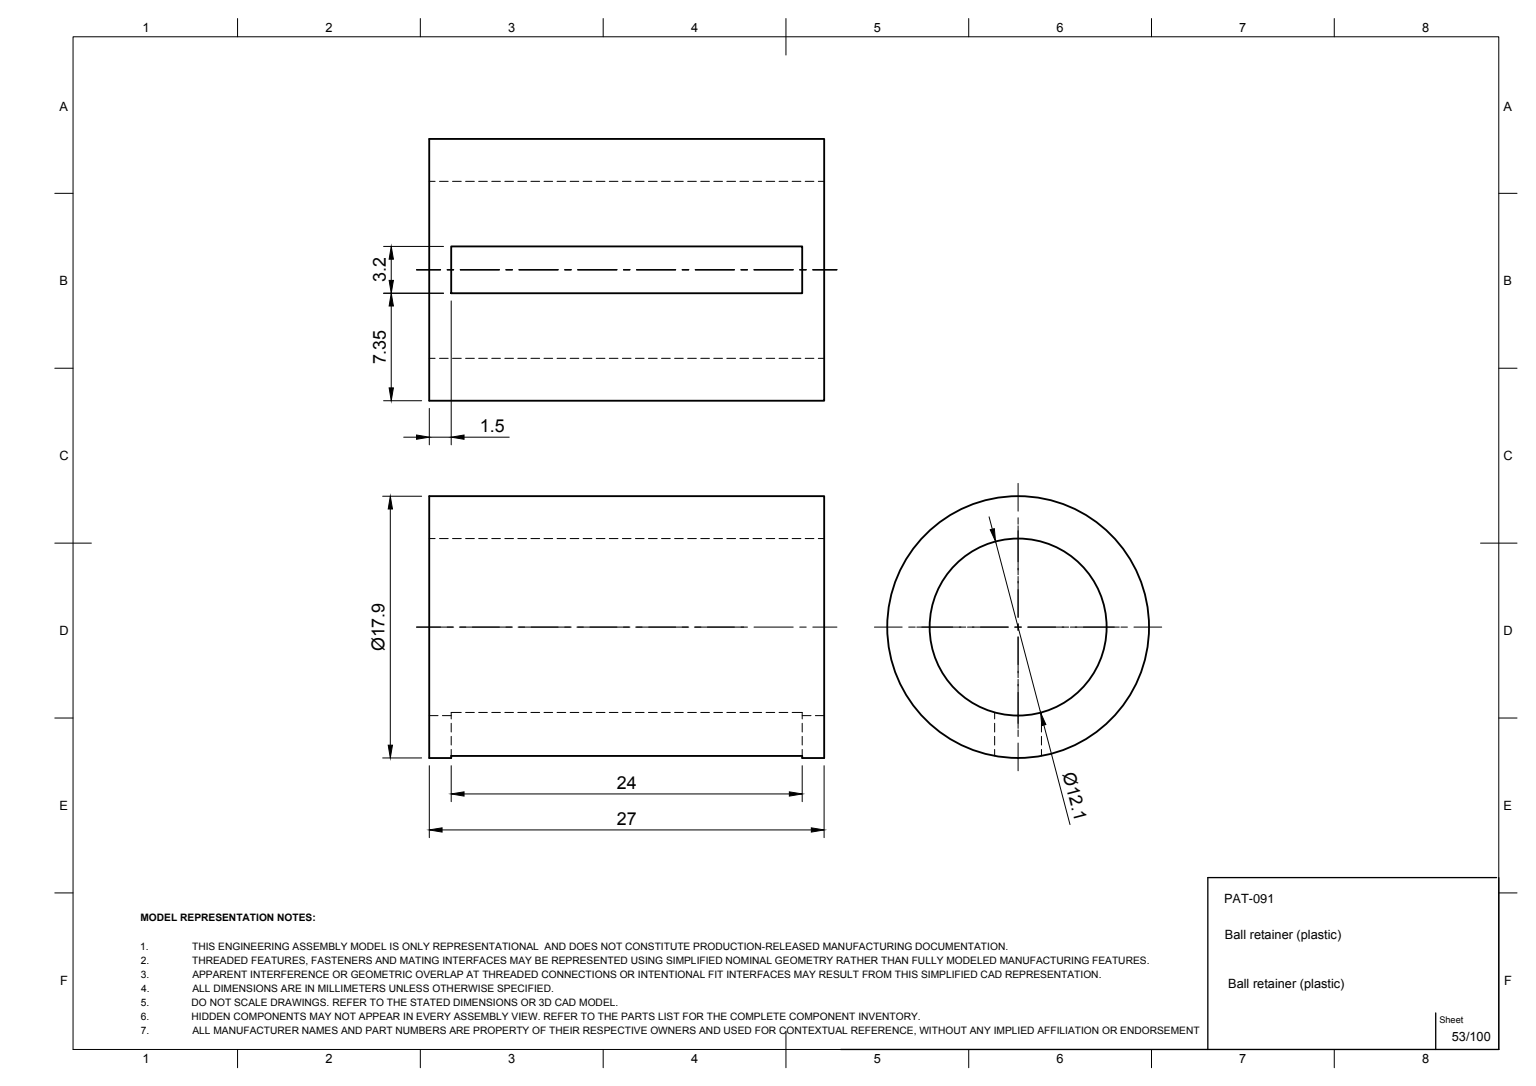
ISO-10303-21;
HEADER;
/* Generated by software containing ST-Developer
 * from STEP Tools, Inc. (www.steptools.com) 
 */

FILE_DESCRIPTION(
/* description */ ('PAT-091'),
/* implementation_level */ '2;1');

FILE_NAME(
/* name */ 'Ball retainer (plastic).step',
/* time_stamp */ '2026-10-27T15:34:44-07:00',
/* author */ (''),
/* organization */ (''),
/* preprocessor_version */ 'ST-DEVELOPER v20.2',
/* originating_system */ 'Autodesk Translation Framework v15.17.0.0',
/* authorisation */ '');

FILE_SCHEMA (('AUTOMOTIVE_DESIGN { 1 0 10303 214 3 1 1 }'));
ENDSEC;

DATA;
#10=MECHANICAL_DESIGN_GEOMETRIC_PRESENTATION_REPRESENTATION('',(#1025),#25100);
#805=SHAPE_REPRESENTATION_RELATIONSHIP('SRR','None',#25570,#915);
#915=ADVANCED_BREP_SHAPE_REPRESENTATION('',(#1147),#25040);
#1025=STYLED_ITEM('',(#26184),#1147);
#1147=MANIFOLD_SOLID_BREP('Body1',#13304);
#1479=FACE_BOUND('',#3579,.T.);
#1480=FACE_BOUND('',#3581,.T.);
#1481=FACE_BOUND('',#3583,.T.);
#1482=FACE_BOUND('',#3585,.T.);
#1880=PLANE('',#15452);
#1881=PLANE('',#15455);
#1882=PLANE('',#15456);
#1883=PLANE('',#15459);
#1884=PLANE('',#15460);
#1885=PLANE('',#15465);
#2492=FACE_OUTER_BOUND('',#3574,.T.);
#2493=FACE_OUTER_BOUND('',#3575,.T.);
#2494=FACE_OUTER_BOUND('',#3576,.T.);
#2495=FACE_OUTER_BOUND('',#3577,.T.);
#2496=FACE_OUTER_BOUND('',#3578,.T.);
#2497=FACE_OUTER_BOUND('',#3580,.T.);
#2498=FACE_OUTER_BOUND('',#3582,.T.);
#2499=FACE_OUTER_BOUND('',#3584,.T.);
#3574=EDGE_LOOP('',(#10692,#10693,#10694,#10695));
#3575=EDGE_LOOP('',(#10696,#10697,#10698,#10699));
#3576=EDGE_LOOP('',(#10700,#10701,#10702,#10703));
#3577=EDGE_LOOP('',(#10704,#10705,#10706,#10707));
#3578=EDGE_LOOP('',(#10708));
#3579=EDGE_LOOP('',(#10709));
#3580=EDGE_LOOP('',(#10710,#10711,#10712,#10713));
#3581=EDGE_LOOP('',(#10714,#10715,#10716,#10717));
#3582=EDGE_LOOP('',(#10718));
#3583=EDGE_LOOP('',(#10719));
#3584=EDGE_LOOP('',(#10720,#10721,#10722,#10723));
#3585=EDGE_LOOP('',(#10724,#10725,#10726,#10727));
#4603=LINE('',#22952,#5343);
#4604=LINE('',#22955,#5344);
#4605=LINE('',#22958,#5345);
#4606=LINE('',#22960,#5346);
#4607=LINE('',#22961,#5347);
#4608=LINE('',#22967,#5348);
#4609=LINE('',#22969,#5349);
#4610=LINE('',#22970,#5350);
#4611=LINE('',#22979,#5351);
#4612=LINE('',#22984,#5352);
#5343=VECTOR('',#18685,1.);
#5344=VECTOR('',#18688,1.);
#5345=VECTOR('',#18691,1.);
#5346=VECTOR('',#18692,1.);
#5347=VECTOR('',#18693,1.);
#5348=VECTOR('',#18700,1.);
#5349=VECTOR('',#18703,1.);
#5350=VECTOR('',#18704,1.);
#5351=VECTOR('',#18715,0.895);
#5352=VECTOR('',#18722,0.605);
#5981=CIRCLE('',#15453,0.895);
#5982=CIRCLE('',#15454,0.605);
#5983=CIRCLE('',#15457,0.895);
#5984=CIRCLE('',#15458,0.605);
#5985=CIRCLE('',#15461,0.895);
#5986=CIRCLE('',#15462,0.605);
#5987=CIRCLE('',#15464,0.895);
#5988=CIRCLE('',#15466,0.605);
#6954=VERTEX_POINT('',#22948);
#6955=VERTEX_POINT('',#22949);
#6956=VERTEX_POINT('',#22951);
#6957=VERTEX_POINT('',#22953);
#6958=VERTEX_POINT('',#22957);
#6959=VERTEX_POINT('',#22959);
#6960=VERTEX_POINT('',#22963);
#6961=VERTEX_POINT('',#22965);
#6962=VERTEX_POINT('',#22972);
#6963=VERTEX_POINT('',#22974);
#6964=VERTEX_POINT('',#22977);
#6965=VERTEX_POINT('',#22981);
#8281=EDGE_CURVE('',#6954,#6955,#5981,.T.);
#8282=EDGE_CURVE('',#6956,#6954,#4603,.T.);
#8283=EDGE_CURVE('',#6957,#6956,#5982,.T.);
#8284=EDGE_CURVE('',#6955,#6957,#4604,.T.);
#8285=EDGE_CURVE('',#6955,#6958,#4605,.T.);
#8286=EDGE_CURVE('',#6959,#6957,#4606,.T.);
#8287=EDGE_CURVE('',#6959,#6958,#4607,.T.);
#8288=EDGE_CURVE('',#6958,#6960,#5983,.T.);
#8289=EDGE_CURVE('',#6961,#6959,#5984,.T.);
#8290=EDGE_CURVE('',#6960,#6961,#4608,.T.);
#8291=EDGE_CURVE('',#6960,#6954,#4609,.T.);
#8292=EDGE_CURVE('',#6956,#6961,#4610,.T.);
#8293=EDGE_CURVE('',#6962,#6962,#5985,.T.);
#8294=EDGE_CURVE('',#6963,#6963,#5986,.T.);
#8295=EDGE_CURVE('',#6964,#6964,#5987,.T.);
#8296=EDGE_CURVE('',#6964,#6962,#4611,.T.);
#8297=EDGE_CURVE('',#6965,#6965,#5988,.T.);
#8298=EDGE_CURVE('',#6965,#6963,#4612,.T.);
#10692=ORIENTED_EDGE('',*,*,#8281,.F.);
#10693=ORIENTED_EDGE('',*,*,#8282,.F.);
#10694=ORIENTED_EDGE('',*,*,#8283,.F.);
#10695=ORIENTED_EDGE('',*,*,#8284,.F.);
#10696=ORIENTED_EDGE('',*,*,#8285,.F.);
#10697=ORIENTED_EDGE('',*,*,#8284,.T.);
#10698=ORIENTED_EDGE('',*,*,#8286,.F.);
#10699=ORIENTED_EDGE('',*,*,#8287,.T.);
#10700=ORIENTED_EDGE('',*,*,#8288,.F.);
#10701=ORIENTED_EDGE('',*,*,#8287,.F.);
#10702=ORIENTED_EDGE('',*,*,#8289,.F.);
#10703=ORIENTED_EDGE('',*,*,#8290,.F.);
#10704=ORIENTED_EDGE('',*,*,#8291,.F.);
#10705=ORIENTED_EDGE('',*,*,#8290,.T.);
#10706=ORIENTED_EDGE('',*,*,#8292,.F.);
#10707=ORIENTED_EDGE('',*,*,#8282,.T.);
#10708=ORIENTED_EDGE('',*,*,#8293,.F.);
#10709=ORIENTED_EDGE('',*,*,#8294,.T.);
#10710=ORIENTED_EDGE('',*,*,#8295,.F.);
#10711=ORIENTED_EDGE('',*,*,#8296,.T.);
#10712=ORIENTED_EDGE('',*,*,#8293,.T.);
#10713=ORIENTED_EDGE('',*,*,#8296,.F.);
#10714=ORIENTED_EDGE('',*,*,#8288,.T.);
#10715=ORIENTED_EDGE('',*,*,#8291,.T.);
#10716=ORIENTED_EDGE('',*,*,#8281,.T.);
#10717=ORIENTED_EDGE('',*,*,#8285,.T.);
#10718=ORIENTED_EDGE('',*,*,#8295,.T.);
#10719=ORIENTED_EDGE('',*,*,#8297,.F.);
#10720=ORIENTED_EDGE('',*,*,#8297,.T.);
#10721=ORIENTED_EDGE('',*,*,#8298,.T.);
#10722=ORIENTED_EDGE('',*,*,#8294,.F.);
#10723=ORIENTED_EDGE('',*,*,#8298,.F.);
#10724=ORIENTED_EDGE('',*,*,#8289,.T.);
#10725=ORIENTED_EDGE('',*,*,#8286,.T.);
#10726=ORIENTED_EDGE('',*,*,#8283,.T.);
#10727=ORIENTED_EDGE('',*,*,#8292,.T.);
#12256=CYLINDRICAL_SURFACE('',#15463,0.895);
#12257=CYLINDRICAL_SURFACE('',#15467,0.605);
#12859=ADVANCED_FACE('',(#2492),#1880,.F.);
#12860=ADVANCED_FACE('',(#2493),#1881,.F.);
#12861=ADVANCED_FACE('',(#2494),#1882,.F.);
#12862=ADVANCED_FACE('',(#2495),#1883,.F.);
#12863=ADVANCED_FACE('',(#2496,#1479),#1884,.T.);
#12864=ADVANCED_FACE('',(#2497,#1480),#12256,.T.);
#12865=ADVANCED_FACE('',(#2498,#1481),#1885,.T.);
#12866=ADVANCED_FACE('',(#2499,#1482),#12257,.F.);
#13304=CLOSED_SHELL('',(#12859,#12860,#12861,#12862,#12863,#12864,#12865,
#12866));
#15451=AXIS2_PLACEMENT_3D('',#22946,#18679,#18680);
#15452=AXIS2_PLACEMENT_3D('',#22947,#18681,#18682);
#15453=AXIS2_PLACEMENT_3D('',#22950,#18683,#18684);
#15454=AXIS2_PLACEMENT_3D('',#22954,#18686,#18687);
#15455=AXIS2_PLACEMENT_3D('',#22956,#18689,#18690);
#15456=AXIS2_PLACEMENT_3D('',#22962,#18694,#18695);
#15457=AXIS2_PLACEMENT_3D('',#22964,#18696,#18697);
#15458=AXIS2_PLACEMENT_3D('',#22966,#18698,#18699);
#15459=AXIS2_PLACEMENT_3D('',#22968,#18701,#18702);
#15460=AXIS2_PLACEMENT_3D('',#22971,#18705,#18706);
#15461=AXIS2_PLACEMENT_3D('',#22973,#18707,#18708);
#15462=AXIS2_PLACEMENT_3D('',#22975,#18709,#18710);
#15463=AXIS2_PLACEMENT_3D('',#22976,#18711,#18712);
#15464=AXIS2_PLACEMENT_3D('',#22978,#18713,#18714);
#15465=AXIS2_PLACEMENT_3D('',#22980,#18716,#18717);
#15466=AXIS2_PLACEMENT_3D('',#22982,#18718,#18719);
#15467=AXIS2_PLACEMENT_3D('',#22983,#18720,#18721);
#18679=DIRECTION('axis',(0.,0.,1.));
#18680=DIRECTION('refdir',(1.,0.,0.));
#18681=DIRECTION('center_axis',(0.,1.,0.));
#18682=DIRECTION('ref_axis',(0.,0.,1.));
#18683=DIRECTION('center_axis',(0.,1.,0.));
#18684=DIRECTION('ref_axis',(1.,0.,0.));
#18685=DIRECTION('',(1.,0.,0.));
#18686=DIRECTION('center_axis',(0.,-1.,0.));
#18687=DIRECTION('ref_axis',(1.,0.,0.));
#18688=DIRECTION('',(-1.,0.,0.));
#18689=DIRECTION('center_axis',(0.,0.,-1.));
#18690=DIRECTION('ref_axis',(-1.,0.,0.));
#18691=DIRECTION('',(0.,-1.,0.));
#18692=DIRECTION('',(0.,1.,0.));
#18693=DIRECTION('',(1.,0.,0.));
#18694=DIRECTION('center_axis',(0.,-1.,0.));
#18695=DIRECTION('ref_axis',(0.,0.,-1.));
#18696=DIRECTION('center_axis',(0.,-1.,0.));
#18697=DIRECTION('ref_axis',(1.,0.,0.));
#18698=DIRECTION('center_axis',(0.,1.,0.));
#18699=DIRECTION('ref_axis',(1.,0.,0.));
#18700=DIRECTION('',(-1.,0.,0.));
#18701=DIRECTION('center_axis',(0.,0.,1.));
#18702=DIRECTION('ref_axis',(1.,0.,0.));
#18703=DIRECTION('',(0.,1.,0.));
#18704=DIRECTION('',(0.,-1.,0.));
#18705=DIRECTION('center_axis',(0.,1.,0.));
#18706=DIRECTION('ref_axis',(0.,0.,1.));
#18707=DIRECTION('center_axis',(0.,-1.,0.));
#18708=DIRECTION('ref_axis',(1.,0.,0.));
#18709=DIRECTION('center_axis',(0.,-1.,0.));
#18710=DIRECTION('ref_axis',(1.,0.,0.));
#18711=DIRECTION('center_axis',(0.,-1.,0.));
#18712=DIRECTION('ref_axis',(1.,0.,0.));
#18713=DIRECTION('center_axis',(0.,-1.,0.));
#18714=DIRECTION('ref_axis',(1.,0.,0.));
#18715=DIRECTION('',(0.,1.,0.));
#18716=DIRECTION('center_axis',(0.,-1.,0.));
#18717=DIRECTION('ref_axis',(0.,0.,-1.));
#18718=DIRECTION('center_axis',(0.,-1.,0.));
#18719=DIRECTION('ref_axis',(1.,0.,0.));
#18720=DIRECTION('center_axis',(0.,-1.,0.));
#18721=DIRECTION('ref_axis',(1.,0.,0.));
#18722=DIRECTION('',(0.,1.,0.));
#22946=CARTESIAN_POINT('',(0.,0.,0.));
#22947=CARTESIAN_POINT('Origin',(0.75,1.2,0.));
#22948=CARTESIAN_POINT('',(0.880582193778639,1.2,0.16));
#22949=CARTESIAN_POINT('',(0.880582193778639,1.2,-0.16));
#22950=CARTESIAN_POINT('Origin',(0.,1.2,0.));
#22951=CARTESIAN_POINT('',(0.583459510163302,1.2,0.16));
#22952=CARTESIAN_POINT('',(0.57,1.2,0.16));
#22953=CARTESIAN_POINT('',(0.583459510163302,1.2,-0.16));
#22954=CARTESIAN_POINT('Origin',(0.,1.2,0.));
#22955=CARTESIAN_POINT('',(0.93,1.2,-0.16));
#22956=CARTESIAN_POINT('Origin',(0.93,0.,-0.16));
#22957=CARTESIAN_POINT('',(0.880582193778639,-1.2,-0.16));
#22958=CARTESIAN_POINT('',(0.880582193778639,0.,-0.16));
#22959=CARTESIAN_POINT('',(0.583459510163302,-1.2,-0.16));
#22960=CARTESIAN_POINT('',(0.583459510163302,0.,-0.16));
#22961=CARTESIAN_POINT('',(0.93,-1.2,-0.16));
#22962=CARTESIAN_POINT('Origin',(0.75,-1.2,0.));
#22963=CARTESIAN_POINT('',(0.880582193778639,-1.2,0.16));
#22964=CARTESIAN_POINT('Origin',(0.,-1.2,0.));
#22965=CARTESIAN_POINT('',(0.583459510163302,-1.2,0.16));
#22966=CARTESIAN_POINT('Origin',(0.,-1.2,0.));
#22967=CARTESIAN_POINT('',(0.57,-1.2,0.16));
#22968=CARTESIAN_POINT('Origin',(0.57,0.,0.16));
#22969=CARTESIAN_POINT('',(0.880582193778639,0.,0.16));
#22970=CARTESIAN_POINT('',(0.583459510163302,0.,0.16));
#22971=CARTESIAN_POINT('Origin',(0.895,1.35,0.));
#22972=CARTESIAN_POINT('',(-0.895,1.35,-1.09605888523688E-16));
#22973=CARTESIAN_POINT('Origin',(0.,1.35,0.));
#22974=CARTESIAN_POINT('',(-0.605,1.35,-7.40911313484149E-17));
#22975=CARTESIAN_POINT('Origin',(0.,1.35,0.));
#22976=CARTESIAN_POINT('Origin',(0.,0.,0.));
#22977=CARTESIAN_POINT('',(-0.895,-1.35,-1.09605888523688E-16));
#22978=CARTESIAN_POINT('Origin',(0.,-1.35,0.));
#22979=CARTESIAN_POINT('',(-0.895,0.,-1.09605888523688E-16));
#22980=CARTESIAN_POINT('Origin',(0.605,-1.35,0.));
#22981=CARTESIAN_POINT('',(-0.605,-1.35,-7.40911313484149E-17));
#22982=CARTESIAN_POINT('Origin',(0.,-1.35,0.));
#22983=CARTESIAN_POINT('Origin',(0.,0.,0.));
#22984=CARTESIAN_POINT('',(-0.605,0.,-7.40911313484149E-17));
#24919=UNCERTAINTY_MEASURE_WITH_UNIT(LENGTH_MEASURE(0.001),#25101,
'DISTANCE_ACCURACY_VALUE',
'Maximum model space distance between geometric entities at asserted c
onnectivities');
#24979=UNCERTAINTY_MEASURE_WITH_UNIT(LENGTH_MEASURE(0.001),#25101,
'DISTANCE_ACCURACY_VALUE',
'Maximum model space distance between geometric entities at asserted c
onnectivities');
#25040=(
GEOMETRIC_REPRESENTATION_CONTEXT(3)
GLOBAL_UNCERTAINTY_ASSIGNED_CONTEXT((#24919))
GLOBAL_UNIT_ASSIGNED_CONTEXT((#25101,#25103,#25104))
REPRESENTATION_CONTEXT('','3D')
);
#25100=(
GEOMETRIC_REPRESENTATION_CONTEXT(3)
GLOBAL_UNCERTAINTY_ASSIGNED_CONTEXT((#24979))
GLOBAL_UNIT_ASSIGNED_CONTEXT((#25101,#25103,#25104))
REPRESENTATION_CONTEXT('','3D')
);
#25101=(
LENGTH_UNIT()
NAMED_UNIT(*)
SI_UNIT(.CENTI.,.METRE.)
);
#25103=(
NAMED_UNIT(*)
PLANE_ANGLE_UNIT()
SI_UNIT($,.RADIAN.)
);
#25104=(
NAMED_UNIT(*)
SI_UNIT($,.STERADIAN.)
SOLID_ANGLE_UNIT()
);
#25165=SHAPE_DEFINITION_REPRESENTATION(#25285,#25570);
#25285=PRODUCT_DEFINITION_SHAPE('',$,#25691);
#25570=SHAPE_REPRESENTATION('',(#15451),#25040);
#25630=PRODUCT_DEFINITION_CONTEXT('part definition',#25992,'design');
#25691=PRODUCT_DEFINITION('Ball retainer (plastic)',
'Ball retainer (plastic)',#25811,#25630);
#25811=PRODUCT_DEFINITION_FORMATION('',$,#26054);
#25992=APPLICATION_CONTEXT(
'Core Data for Automotive Mechanical Design Process');
#25993=PRODUCT_CONTEXT('part definition',#25992,'mechanical');
#26054=PRODUCT('Ball retainer (plastic)','Ball retainer (plastic)',
'Ball retainer (plastic)',(#25993));
#26178=COLOUR_RGB('Sky Blue',0.24,0.69,0.87);
#26179=FILL_AREA_STYLE_COLOUR('',#26178);
#26180=FILL_AREA_STYLE('',(#26179));
#26181=SURFACE_STYLE_FILL_AREA(#26180);
#26182=SURFACE_SIDE_STYLE('',(#26181));
#26183=SURFACE_STYLE_USAGE(.BOTH.,#26182);
#26184=PRESENTATION_STYLE_ASSIGNMENT((#26183));
ENDSEC;
END-ISO-10303-21;
